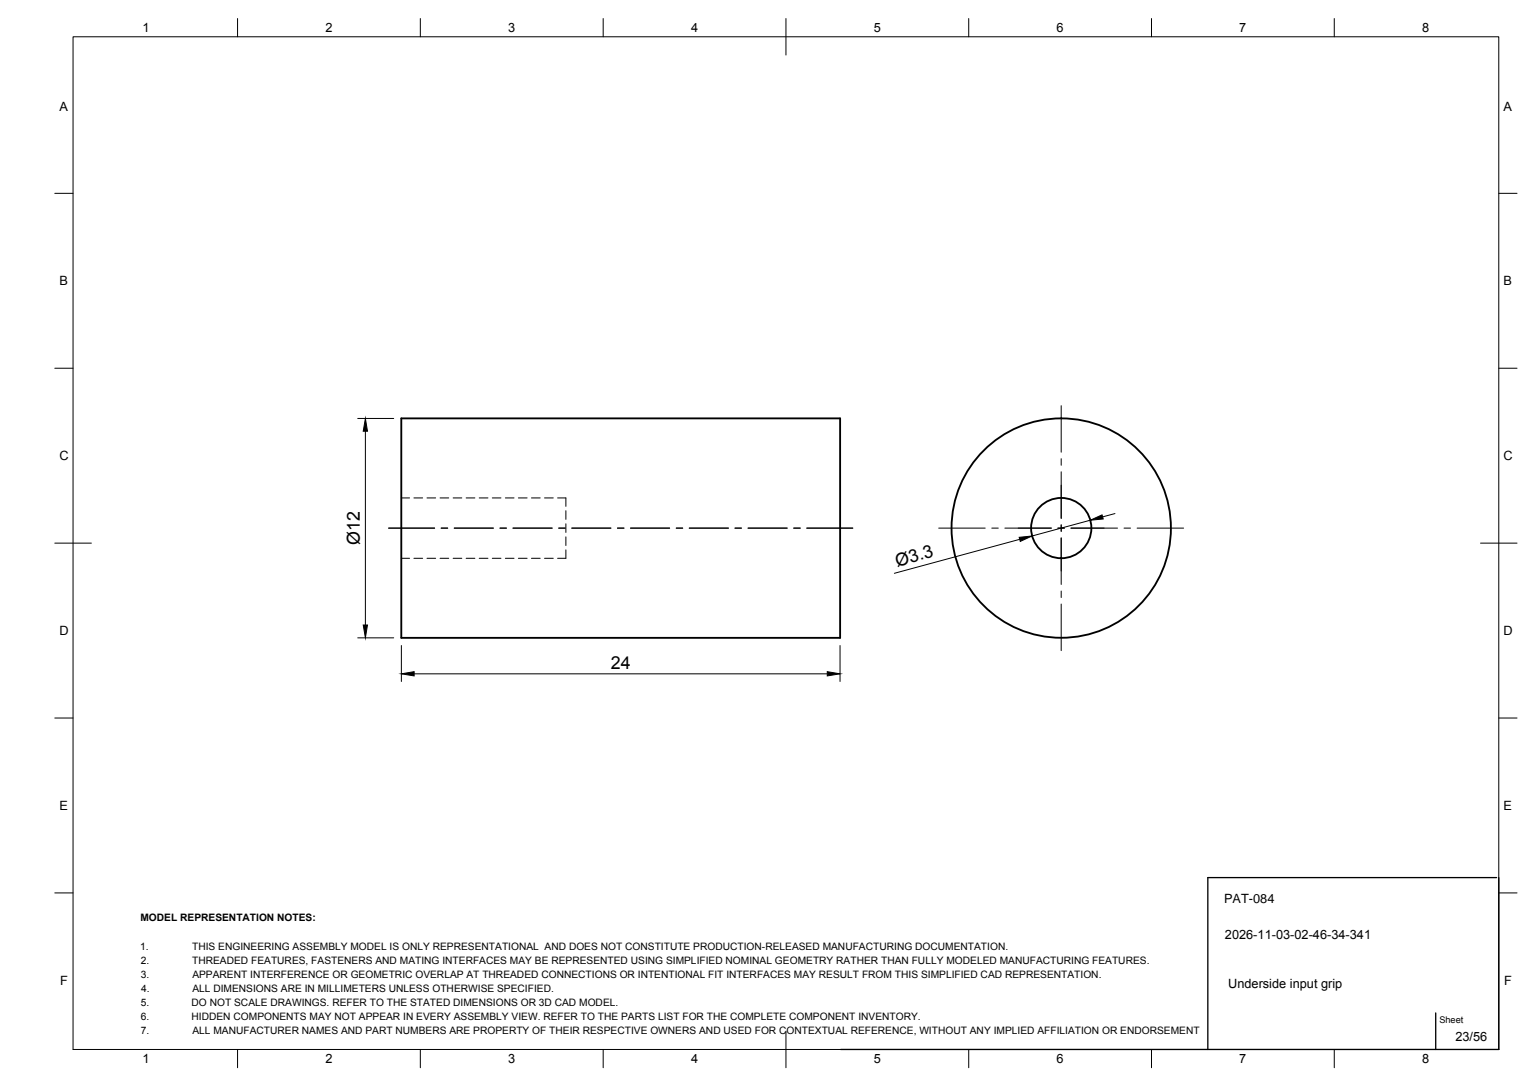
ISO-10303-21;
HEADER;
/* Generated by software containing ST-Developer
 * from STEP Tools, Inc. (www.steptools.com) 
 */

FILE_DESCRIPTION(
/* description */ ('Quick-return (Whitworth) mechanism'),
/* implementation_level */ '2;1');

FILE_NAME(
/* name */ 'Underside input grip.step',
/* time_stamp */ '2026-10-28T03:25:57-07:00',
/* author */ (''),
/* organization */ (''),
/* preprocessor_version */ 'ST-DEVELOPER v20.2',
/* originating_system */ 'Autodesk Translation Framework v15.17.0.0',
/* authorisation */ '');

FILE_SCHEMA (('AUTOMOTIVE_DESIGN { 1 0 10303 214 3 1 1 }'));
ENDSEC;

DATA;
#10=MECHANICAL_DESIGN_GEOMETRIC_PRESENTATION_REPRESENTATION('',(#512),#14878);
#416=SHAPE_REPRESENTATION_RELATIONSHIP('SRR','None',#15086,#460);
#460=ADVANCED_BREP_SHAPE_REPRESENTATION('',(#564),#14843);
#512=STYLED_ITEM('',(#15413),#564);
#564=MANIFOLD_SOLID_BREP('Body1',#7866);
#708=FACE_BOUND('',#1851,.T.);
#881=PLANE('',#8880);
#882=PLANE('',#8884);
#883=PLANE('',#8885);
#1264=FACE_OUTER_BOUND('',#1847,.T.);
#1265=FACE_OUTER_BOUND('',#1848,.T.);
#1266=FACE_OUTER_BOUND('',#1849,.T.);
#1267=FACE_OUTER_BOUND('',#1850,.T.);
#1268=FACE_OUTER_BOUND('',#1852,.T.);
#1847=EDGE_LOOP('',(#6202,#6203,#6204,#6205));
#1848=EDGE_LOOP('',(#6206));
#1849=EDGE_LOOP('',(#6207,#6208,#6209,#6210));
#1850=EDGE_LOOP('',(#6211));
#1851=EDGE_LOOP('',(#6212));
#1852=EDGE_LOOP('',(#6213));
#2362=LINE('',#13459,#2885);
#2363=LINE('',#13466,#2886);
#2885=VECTOR('',#10579,0.165);
#2886=VECTOR('',#10588,0.6);
#3468=CIRCLE('',#8878,0.165);
#3469=CIRCLE('',#8879,0.165);
#3470=CIRCLE('',#8882,0.6);
#3471=CIRCLE('',#8883,0.6);
#3955=VERTEX_POINT('',#13456);
#3956=VERTEX_POINT('',#13458);
#3957=VERTEX_POINT('',#13463);
#3958=VERTEX_POINT('',#13465);
#4758=EDGE_CURVE('',#3955,#3955,#3468,.T.);
#4759=EDGE_CURVE('',#3955,#3956,#2362,.T.);
#4760=EDGE_CURVE('',#3956,#3956,#3469,.T.);
#4761=EDGE_CURVE('',#3957,#3957,#3470,.T.);
#4762=EDGE_CURVE('',#3957,#3958,#2363,.T.);
#4763=EDGE_CURVE('',#3958,#3958,#3471,.T.);
#6202=ORIENTED_EDGE('',*,*,#4758,.F.);
#6203=ORIENTED_EDGE('',*,*,#4759,.T.);
#6204=ORIENTED_EDGE('',*,*,#4760,.F.);
#6205=ORIENTED_EDGE('',*,*,#4759,.F.);
#6206=ORIENTED_EDGE('',*,*,#4758,.T.);
#6207=ORIENTED_EDGE('',*,*,#4761,.F.);
#6208=ORIENTED_EDGE('',*,*,#4762,.T.);
#6209=ORIENTED_EDGE('',*,*,#4763,.T.);
#6210=ORIENTED_EDGE('',*,*,#4762,.F.);
#6211=ORIENTED_EDGE('',*,*,#4761,.T.);
#6212=ORIENTED_EDGE('',*,*,#4760,.T.);
#6213=ORIENTED_EDGE('',*,*,#4763,.F.);
#7306=CYLINDRICAL_SURFACE('',#8877,0.165);
#7307=CYLINDRICAL_SURFACE('',#8881,0.6);
#7595=ADVANCED_FACE('',(#1264),#7306,.F.);
#7596=ADVANCED_FACE('',(#1265),#881,.T.);
#7597=ADVANCED_FACE('',(#1266),#7307,.T.);
#7598=ADVANCED_FACE('',(#1267,#708),#882,.T.);
#7599=ADVANCED_FACE('',(#1268),#883,.F.);
#7866=CLOSED_SHELL('',(#7595,#7596,#7597,#7598,#7599));
#8876=AXIS2_PLACEMENT_3D('',#13454,#10573,#10574);
#8877=AXIS2_PLACEMENT_3D('',#13455,#10575,#10576);
#8878=AXIS2_PLACEMENT_3D('',#13457,#10577,#10578);
#8879=AXIS2_PLACEMENT_3D('',#13460,#10580,#10581);
#8880=AXIS2_PLACEMENT_3D('',#13461,#10582,#10583);
#8881=AXIS2_PLACEMENT_3D('',#13462,#10584,#10585);
#8882=AXIS2_PLACEMENT_3D('',#13464,#10586,#10587);
#8883=AXIS2_PLACEMENT_3D('',#13467,#10589,#10590);
#8884=AXIS2_PLACEMENT_3D('',#13468,#10591,#10592);
#8885=AXIS2_PLACEMENT_3D('',#13469,#10593,#10594);
#10573=DIRECTION('axis',(0.,0.,1.));
#10574=DIRECTION('refdir',(1.,0.,0.));
#10575=DIRECTION('center_axis',(0.,0.,1.));
#10576=DIRECTION('ref_axis',(1.,0.,0.));
#10577=DIRECTION('center_axis',(0.,0.,1.));
#10578=DIRECTION('ref_axis',(1.,0.,0.));
#10579=DIRECTION('',(0.,0.,1.));
#10580=DIRECTION('center_axis',(0.,0.,-1.));
#10581=DIRECTION('ref_axis',(1.,0.,0.));
#10582=DIRECTION('center_axis',(0.,0.,1.));
#10583=DIRECTION('ref_axis',(1.,0.,0.));
#10584=DIRECTION('center_axis',(0.,0.,1.));
#10585=DIRECTION('ref_axis',(1.,0.,0.));
#10586=DIRECTION('center_axis',(0.,0.,1.));
#10587=DIRECTION('ref_axis',(1.,0.,0.));
#10588=DIRECTION('',(0.,0.,-1.));
#10589=DIRECTION('center_axis',(0.,0.,1.));
#10590=DIRECTION('ref_axis',(1.,0.,0.));
#10591=DIRECTION('center_axis',(0.,0.,1.));
#10592=DIRECTION('ref_axis',(1.,0.,0.));
#10593=DIRECTION('center_axis',(0.,0.,1.));
#10594=DIRECTION('ref_axis',(1.,0.,0.));
#13454=CARTESIAN_POINT('',(0.,0.,0.));
#13455=CARTESIAN_POINT('Origin',(-3.2,6.,3.9));
#13456=CARTESIAN_POINT('',(-3.365,6.,3.9));
#13457=CARTESIAN_POINT('Origin',(-3.2,6.,3.9));
#13458=CARTESIAN_POINT('',(-3.365,6.,4.8));
#13459=CARTESIAN_POINT('',(-3.365,6.,3.9));
#13460=CARTESIAN_POINT('Origin',(-3.2,6.,4.8));
#13461=CARTESIAN_POINT('Origin',(-3.2,6.,3.9));
#13462=CARTESIAN_POINT('Origin',(-3.2,6.,2.4));
#13463=CARTESIAN_POINT('',(-3.8,6.,4.8));
#13464=CARTESIAN_POINT('Origin',(-3.2,6.,4.8));
#13465=CARTESIAN_POINT('',(-3.8,6.,2.4));
#13466=CARTESIAN_POINT('',(-3.8,6.,2.4));
#13467=CARTESIAN_POINT('Origin',(-3.2,6.,2.4));
#13468=CARTESIAN_POINT('Origin',(-3.2,6.,4.8));
#13469=CARTESIAN_POINT('Origin',(-3.2,6.,2.4));
#14789=UNCERTAINTY_MEASURE_WITH_UNIT(LENGTH_MEASURE(0.001),#14879,
'DISTANCE_ACCURACY_VALUE',
'Maximum model space distance between geometric entities at asserted c
onnectivities');
#14824=UNCERTAINTY_MEASURE_WITH_UNIT(LENGTH_MEASURE(0.001),#14879,
'DISTANCE_ACCURACY_VALUE',
'Maximum model space distance between geometric entities at asserted c
onnectivities');
#14843=(
GEOMETRIC_REPRESENTATION_CONTEXT(3)
GLOBAL_UNCERTAINTY_ASSIGNED_CONTEXT((#14789))
GLOBAL_UNIT_ASSIGNED_CONTEXT((#14879,#14881,#14882))
REPRESENTATION_CONTEXT('','3D')
);
#14878=(
GEOMETRIC_REPRESENTATION_CONTEXT(3)
GLOBAL_UNCERTAINTY_ASSIGNED_CONTEXT((#14824))
GLOBAL_UNIT_ASSIGNED_CONTEXT((#14879,#14881,#14882))
REPRESENTATION_CONTEXT('','3D')
);
#14879=(
LENGTH_UNIT()
NAMED_UNIT(*)
SI_UNIT(.CENTI.,.METRE.)
);
#14881=(
NAMED_UNIT(*)
PLANE_ANGLE_UNIT()
SI_UNIT($,.RADIAN.)
);
#14882=(
NAMED_UNIT(*)
SI_UNIT($,.STERADIAN.)
SOLID_ANGLE_UNIT()
);
#14901=SHAPE_DEFINITION_REPRESENTATION(#14959,#15086);
#14959=PRODUCT_DEFINITION_SHAPE('',$,#15140);
#15086=SHAPE_REPRESENTATION('',(#8876),#14843);
#15121=PRODUCT_DEFINITION_CONTEXT('part definition',#15282,'design');
#15140=PRODUCT_DEFINITION('Underside input grip','Underside input grip',
#15193,#15121);
#15193=PRODUCT_DEFINITION_FORMATION('',$,#15302);
#15282=APPLICATION_CONTEXT(
'Core Data for Automotive Mechanical Design Process');
#15283=PRODUCT_CONTEXT('part definition',#15282,'mechanical');
#15302=PRODUCT('Underside input grip','Underside input grip',
'Underside input grip',(#15283));
#15407=COLOUR_RGB('Black',0.12,0.14,0.17);
#15408=FILL_AREA_STYLE_COLOUR('',#15407);
#15409=FILL_AREA_STYLE('',(#15408));
#15410=SURFACE_STYLE_FILL_AREA(#15409);
#15411=SURFACE_SIDE_STYLE('',(#15410));
#15412=SURFACE_STYLE_USAGE(.BOTH.,#15411);
#15413=PRESENTATION_STYLE_ASSIGNMENT((#15412));
ENDSEC;
END-ISO-10303-21;
